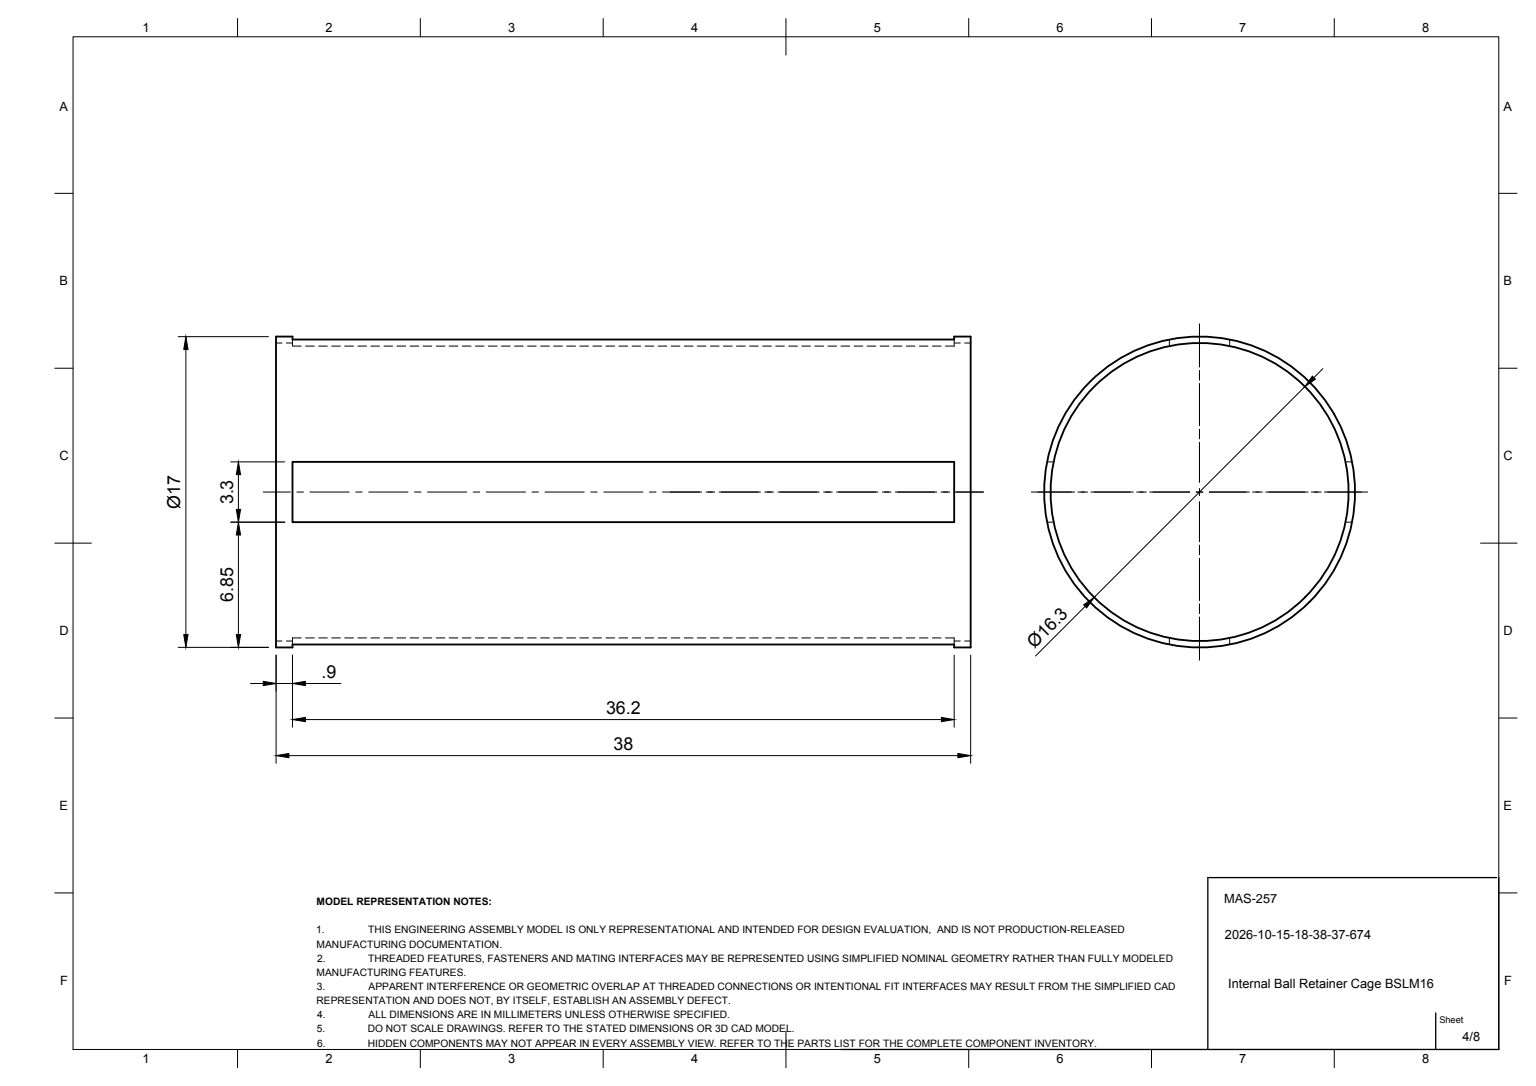
ISO-10303-21;
HEADER;
FILE_DESCRIPTION((''),'2;1');
FILE_NAME('Internal Ball Retainer Cage BSLM16.step','2026-10-05T22:33:56+05:00',(''),(''),'','','');
FILE_SCHEMA (('AUTOMOTIVE_DESIGN { 1 0 10303 214 3 1 1 }'));
ENDSEC;
DATA;
#10=MECHANICAL_DESIGN_GEOMETRIC_PRESENTATION_REPRESENTATION('',(#431),#16942);
#417=SHAPE_REPRESENTATION_RELATIONSHIP('SRR','None',#17021,#424) ;
#424=ADVANCED_BREP_SHAPE_REPRESENTATION('',(#438),#16937) ;
#431=STYLED_ITEM('',(#17065),#438) ;
#438=MANIFOLD_SOLID_BREP('Internal Ball Retainer Cage BSLM16',#8180) ;
#719=FACE_BOUND('',#1778,.T.) ;
#720=FACE_BOUND('',#1779,.T.) ;
#721=FACE_BOUND('',#1780,.T.) ;
#722=FACE_BOUND('',#1781,.T.) ;
#723=FACE_BOUND('',#1783,.T.) ;
#724=FACE_BOUND('',#1785,.T.) ;
#725=FACE_BOUND('',#1786,.T.) ;
#726=FACE_BOUND('',#1787,.T.) ;
#727=FACE_BOUND('',#1788,.T.) ;
#728=FACE_BOUND('',#1790,.T.) ;
#818=PLANE('',#8553) ;
#819=PLANE('',#8554) ;
#820=PLANE('',#8557) ;
#821=PLANE('',#8558) ;
#822=PLANE('',#8561) ;
#823=PLANE('',#8562) ;
#824=PLANE('',#8565) ;
#825=PLANE('',#8566) ;
#826=PLANE('',#8569) ;
#827=PLANE('',#8570) ;
#828=PLANE('',#8573) ;
#829=PLANE('',#8574) ;
#830=PLANE('',#8577) ;
#831=PLANE('',#8578) ;
#832=PLANE('',#8581) ;
#833=PLANE('',#8582) ;
#834=PLANE('',#8588) ;
#835=PLANE('',#8592) ;
#1016=CYLINDRICAL_SURFACE('',#8585,8.15) ;
#1017=CYLINDRICAL_SURFACE('',#8590,8.5) ;
#1286=FACE_OUTER_BOUND('',#1761,.T.) ;
#1287=FACE_OUTER_BOUND('',#1762,.T.) ;
#1288=FACE_OUTER_BOUND('',#1763,.T.) ;
#1289=FACE_OUTER_BOUND('',#1764,.T.) ;
#1290=FACE_OUTER_BOUND('',#1765,.T.) ;
#1291=FACE_OUTER_BOUND('',#1766,.T.) ;
#1292=FACE_OUTER_BOUND('',#1767,.T.) ;
#1293=FACE_OUTER_BOUND('',#1768,.T.) ;
#1294=FACE_OUTER_BOUND('',#1769,.T.) ;
#1295=FACE_OUTER_BOUND('',#1770,.T.) ;
#1296=FACE_OUTER_BOUND('',#1771,.T.) ;
#1297=FACE_OUTER_BOUND('',#1772,.T.) ;
#1298=FACE_OUTER_BOUND('',#1773,.T.) ;
#1299=FACE_OUTER_BOUND('',#1774,.T.) ;
#1300=FACE_OUTER_BOUND('',#1775,.T.) ;
#1301=FACE_OUTER_BOUND('',#1776,.T.) ;
#1302=FACE_OUTER_BOUND('',#1777,.T.) ;
#1303=FACE_OUTER_BOUND('',#1782,.T.) ;
#1304=FACE_OUTER_BOUND('',#1784,.T.) ;
#1305=FACE_OUTER_BOUND('',#1789,.T.) ;
#1761=EDGE_LOOP('',(#6517,#6518,#6519,#6520)) ;
#1762=EDGE_LOOP('',(#6521,#6522,#6523,#6524)) ;
#1763=EDGE_LOOP('',(#6525,#6526,#6527,#6528)) ;
#1764=EDGE_LOOP('',(#6529,#6530,#6531,#6532)) ;
#1765=EDGE_LOOP('',(#6533,#6534,#6535,#6536)) ;
#1766=EDGE_LOOP('',(#6537,#6538,#6539,#6540)) ;
#1767=EDGE_LOOP('',(#6541,#6542,#6543,#6544)) ;
#1768=EDGE_LOOP('',(#6545,#6546,#6547,#6548)) ;
#1769=EDGE_LOOP('',(#6549,#6550,#6551,#6552)) ;
#1770=EDGE_LOOP('',(#6553,#6554,#6555,#6556)) ;
#1771=EDGE_LOOP('',(#6557,#6558,#6559,#6560)) ;
#1772=EDGE_LOOP('',(#6561,#6562,#6563,#6564)) ;
#1773=EDGE_LOOP('',(#6565,#6566,#6567,#6568)) ;
#1774=EDGE_LOOP('',(#6569,#6570,#6571,#6572)) ;
#1775=EDGE_LOOP('',(#6573,#6574,#6575,#6576)) ;
#1776=EDGE_LOOP('',(#6577,#6578,#6579,#6580)) ;
#1777=EDGE_LOOP('',(#6581,#6582,#6583,#6584)) ;
#1778=EDGE_LOOP('',(#6585,#6586,#6587,#6588)) ;
#1779=EDGE_LOOP('',(#6589,#6590,#6591,#6592)) ;
#1780=EDGE_LOOP('',(#6593,#6594,#6595,#6596)) ;
#1781=EDGE_LOOP('',(#6597,#6598,#6599,#6600)) ;
#1782=EDGE_LOOP('',(#6601)) ;
#1783=EDGE_LOOP('',(#6602)) ;
#1784=EDGE_LOOP('',(#6603,#6604,#6605,#6606)) ;
#1785=EDGE_LOOP('',(#6607,#6608,#6609,#6610)) ;
#1786=EDGE_LOOP('',(#6611,#6612,#6613,#6614)) ;
#1787=EDGE_LOOP('',(#6615,#6616,#6617,#6618)) ;
#1788=EDGE_LOOP('',(#6619,#6620,#6621,#6622)) ;
#1789=EDGE_LOOP('',(#6623)) ;
#1790=EDGE_LOOP('',(#6624)) ;
#2253=LINE('',#13606,#2815) ;
#2254=LINE('',#13608,#2816) ;
#2255=LINE('',#13610,#2817) ;
#2256=LINE('',#13611,#2818) ;
#2257=LINE('',#13617,#2819) ;
#2258=LINE('',#13620,#2820) ;
#2259=LINE('',#13622,#2821) ;
#2260=LINE('',#13623,#2822) ;
#2261=LINE('',#13630,#2823) ;
#2262=LINE('',#13632,#2824) ;
#2263=LINE('',#13634,#2825) ;
#2264=LINE('',#13635,#2826) ;
#2265=LINE('',#13641,#2827) ;
#2266=LINE('',#13644,#2828) ;
#2267=LINE('',#13646,#2829) ;
#2268=LINE('',#13647,#2830) ;
#2269=LINE('',#13654,#2831) ;
#2270=LINE('',#13656,#2832) ;
#2271=LINE('',#13658,#2833) ;
#2272=LINE('',#13659,#2834) ;
#2273=LINE('',#13665,#2835) ;
#2274=LINE('',#13668,#2836) ;
#2275=LINE('',#13670,#2837) ;
#2276=LINE('',#13671,#2838) ;
#2277=LINE('',#13678,#2839) ;
#2278=LINE('',#13680,#2840) ;
#2279=LINE('',#13682,#2841) ;
#2280=LINE('',#13683,#2842) ;
#2281=LINE('',#13689,#2843) ;
#2282=LINE('',#13692,#2844) ;
#2283=LINE('',#13694,#2845) ;
#2284=LINE('',#13695,#2846) ;
#2285=LINE('',#13703,#2847) ;
#2286=LINE('',#13711,#2848) ;
#2815=VECTOR('',#9811,10.) ;
#2816=VECTOR('',#9812,10.) ;
#2817=VECTOR('',#9813,10.) ;
#2818=VECTOR('',#9814,10.) ;
#2819=VECTOR('',#9821,10.) ;
#2820=VECTOR('',#9824,10.) ;
#2821=VECTOR('',#9825,10.) ;
#2822=VECTOR('',#9826,10.) ;
#2823=VECTOR('',#9835,10.) ;
#2824=VECTOR('',#9836,10.) ;
#2825=VECTOR('',#9837,10.) ;
#2826=VECTOR('',#9838,10.) ;
#2827=VECTOR('',#9845,10.) ;
#2828=VECTOR('',#9848,10.) ;
#2829=VECTOR('',#9849,10.) ;
#2830=VECTOR('',#9850,10.) ;
#2831=VECTOR('',#9859,10.) ;
#2832=VECTOR('',#9860,10.) ;
#2833=VECTOR('',#9861,10.) ;
#2834=VECTOR('',#9862,10.) ;
#2835=VECTOR('',#9869,10.) ;
#2836=VECTOR('',#9872,10.) ;
#2837=VECTOR('',#9873,10.) ;
#2838=VECTOR('',#9874,10.) ;
#2839=VECTOR('',#9883,10.) ;
#2840=VECTOR('',#9884,10.) ;
#2841=VECTOR('',#9885,10.) ;
#2842=VECTOR('',#9886,10.) ;
#2843=VECTOR('',#9893,10.) ;
#2844=VECTOR('',#9896,10.) ;
#2845=VECTOR('',#9897,10.) ;
#2846=VECTOR('',#9898,10.) ;
#2847=VECTOR('',#9909,8.15) ;
#2848=VECTOR('',#9920,8.5) ;
#3253=CIRCLE('',#8555,8.15) ;
#3254=CIRCLE('',#8556,8.5) ;
#3255=CIRCLE('',#8559,8.15) ;
#3256=CIRCLE('',#8560,8.5) ;
#3257=CIRCLE('',#8563,8.15) ;
#3258=CIRCLE('',#8564,8.5) ;
#3259=CIRCLE('',#8567,8.15) ;
#3260=CIRCLE('',#8568,8.5) ;
#3261=CIRCLE('',#8571,8.15) ;
#3262=CIRCLE('',#8572,8.5) ;
#3263=CIRCLE('',#8575,8.15) ;
#3264=CIRCLE('',#8576,8.5) ;
#3265=CIRCLE('',#8579,8.15) ;
#3266=CIRCLE('',#8580,8.5) ;
#3267=CIRCLE('',#8583,8.15) ;
#3268=CIRCLE('',#8584,8.5) ;
#3269=CIRCLE('',#8586,8.15) ;
#3270=CIRCLE('',#8587,8.15) ;
#3271=CIRCLE('',#8589,8.5) ;
#3272=CIRCLE('',#8591,8.5) ;
#3783=VERTEX_POINT('',#13604) ;
#3784=VERTEX_POINT('',#13605) ;
#3785=VERTEX_POINT('',#13607) ;
#3786=VERTEX_POINT('',#13609) ;
#3787=VERTEX_POINT('',#13613) ;
#3788=VERTEX_POINT('',#13615) ;
#3789=VERTEX_POINT('',#13619) ;
#3790=VERTEX_POINT('',#13621) ;
#3791=VERTEX_POINT('',#13628) ;
#3792=VERTEX_POINT('',#13629) ;
#3793=VERTEX_POINT('',#13631) ;
#3794=VERTEX_POINT('',#13633) ;
#3795=VERTEX_POINT('',#13637) ;
#3796=VERTEX_POINT('',#13639) ;
#3797=VERTEX_POINT('',#13643) ;
#3798=VERTEX_POINT('',#13645) ;
#3799=VERTEX_POINT('',#13652) ;
#3800=VERTEX_POINT('',#13653) ;
#3801=VERTEX_POINT('',#13655) ;
#3802=VERTEX_POINT('',#13657) ;
#3803=VERTEX_POINT('',#13661) ;
#3804=VERTEX_POINT('',#13663) ;
#3805=VERTEX_POINT('',#13667) ;
#3806=VERTEX_POINT('',#13669) ;
#3807=VERTEX_POINT('',#13676) ;
#3808=VERTEX_POINT('',#13677) ;
#3809=VERTEX_POINT('',#13679) ;
#3810=VERTEX_POINT('',#13681) ;
#3811=VERTEX_POINT('',#13685) ;
#3812=VERTEX_POINT('',#13687) ;
#3813=VERTEX_POINT('',#13691) ;
#3814=VERTEX_POINT('',#13693) ;
#3815=VERTEX_POINT('',#13700) ;
#3816=VERTEX_POINT('',#13702) ;
#3817=VERTEX_POINT('',#13706) ;
#3818=VERTEX_POINT('',#13709) ;
#4756=EDGE_CURVE('',#3783,#3784,#2253,.T.) ;
#4757=EDGE_CURVE('',#3783,#3785,#2254,.T.) ;
#4758=EDGE_CURVE('',#3786,#3785,#2255,.T.) ;
#4759=EDGE_CURVE('',#3786,#3784,#2256,.T.) ;
#4760=EDGE_CURVE('',#3784,#3787,#3253,.T.) ;
#4761=EDGE_CURVE('',#3788,#3786,#3254,.T.) ;
#4762=EDGE_CURVE('',#3787,#3788,#2257,.T.) ;
#4763=EDGE_CURVE('',#3787,#3789,#2258,.T.) ;
#4764=EDGE_CURVE('',#3790,#3788,#2259,.T.) ;
#4765=EDGE_CURVE('',#3790,#3789,#2260,.T.) ;
#4766=EDGE_CURVE('',#3789,#3783,#3255,.T.) ;
#4767=EDGE_CURVE('',#3785,#3790,#3256,.T.) ;
#4768=EDGE_CURVE('',#3791,#3792,#2261,.T.) ;
#4769=EDGE_CURVE('',#3791,#3793,#2262,.T.) ;
#4770=EDGE_CURVE('',#3794,#3793,#2263,.T.) ;
#4771=EDGE_CURVE('',#3794,#3792,#2264,.T.) ;
#4772=EDGE_CURVE('',#3792,#3795,#3257,.T.) ;
#4773=EDGE_CURVE('',#3796,#3794,#3258,.T.) ;
#4774=EDGE_CURVE('',#3795,#3796,#2265,.T.) ;
#4775=EDGE_CURVE('',#3795,#3797,#2266,.T.) ;
#4776=EDGE_CURVE('',#3798,#3796,#2267,.T.) ;
#4777=EDGE_CURVE('',#3798,#3797,#2268,.T.) ;
#4778=EDGE_CURVE('',#3797,#3791,#3259,.T.) ;
#4779=EDGE_CURVE('',#3793,#3798,#3260,.T.) ;
#4780=EDGE_CURVE('',#3799,#3800,#2269,.T.) ;
#4781=EDGE_CURVE('',#3799,#3801,#2270,.T.) ;
#4782=EDGE_CURVE('',#3802,#3801,#2271,.T.) ;
#4783=EDGE_CURVE('',#3802,#3800,#2272,.T.) ;
#4784=EDGE_CURVE('',#3800,#3803,#3261,.T.) ;
#4785=EDGE_CURVE('',#3804,#3802,#3262,.T.) ;
#4786=EDGE_CURVE('',#3803,#3804,#2273,.T.) ;
#4787=EDGE_CURVE('',#3803,#3805,#2274,.T.) ;
#4788=EDGE_CURVE('',#3806,#3804,#2275,.T.) ;
#4789=EDGE_CURVE('',#3806,#3805,#2276,.T.) ;
#4790=EDGE_CURVE('',#3805,#3799,#3263,.T.) ;
#4791=EDGE_CURVE('',#3801,#3806,#3264,.T.) ;
#4792=EDGE_CURVE('',#3807,#3808,#2277,.T.) ;
#4793=EDGE_CURVE('',#3807,#3809,#2278,.T.) ;
#4794=EDGE_CURVE('',#3810,#3809,#2279,.T.) ;
#4795=EDGE_CURVE('',#3810,#3808,#2280,.T.) ;
#4796=EDGE_CURVE('',#3808,#3811,#3265,.T.) ;
#4797=EDGE_CURVE('',#3812,#3810,#3266,.T.) ;
#4798=EDGE_CURVE('',#3811,#3812,#2281,.T.) ;
#4799=EDGE_CURVE('',#3811,#3813,#2282,.T.) ;
#4800=EDGE_CURVE('',#3814,#3812,#2283,.T.) ;
#4801=EDGE_CURVE('',#3814,#3813,#2284,.T.) ;
#4802=EDGE_CURVE('',#3813,#3807,#3267,.T.) ;
#4803=EDGE_CURVE('',#3809,#3814,#3268,.T.) ;
#4804=EDGE_CURVE('',#3815,#3815,#3269,.T.) ;
#4805=EDGE_CURVE('',#3815,#3816,#2285,.T.) ;
#4806=EDGE_CURVE('',#3816,#3816,#3270,.T.) ;
#4807=EDGE_CURVE('',#3817,#3817,#3271,.T.) ;
#4808=EDGE_CURVE('',#3818,#3818,#3272,.T.) ;
#4809=EDGE_CURVE('',#3818,#3817,#2286,.T.) ;
#6517=ORIENTED_EDGE('',*,*,#4756,.F.) ;
#6518=ORIENTED_EDGE('',*,*,#4757,.T.) ;
#6519=ORIENTED_EDGE('',*,*,#4758,.F.) ;
#6520=ORIENTED_EDGE('',*,*,#4759,.T.) ;
#6521=ORIENTED_EDGE('',*,*,#4760,.F.) ;
#6522=ORIENTED_EDGE('',*,*,#4759,.F.) ;
#6523=ORIENTED_EDGE('',*,*,#4761,.F.) ;
#6524=ORIENTED_EDGE('',*,*,#4762,.F.) ;
#6525=ORIENTED_EDGE('',*,*,#4763,.F.) ;
#6526=ORIENTED_EDGE('',*,*,#4762,.T.) ;
#6527=ORIENTED_EDGE('',*,*,#4764,.F.) ;
#6528=ORIENTED_EDGE('',*,*,#4765,.T.) ;
#6529=ORIENTED_EDGE('',*,*,#4766,.F.) ;
#6530=ORIENTED_EDGE('',*,*,#4765,.F.) ;
#6531=ORIENTED_EDGE('',*,*,#4767,.F.) ;
#6532=ORIENTED_EDGE('',*,*,#4757,.F.) ;
#6533=ORIENTED_EDGE('',*,*,#4768,.F.) ;
#6534=ORIENTED_EDGE('',*,*,#4769,.T.) ;
#6535=ORIENTED_EDGE('',*,*,#4770,.F.) ;
#6536=ORIENTED_EDGE('',*,*,#4771,.T.) ;
#6537=ORIENTED_EDGE('',*,*,#4772,.F.) ;
#6538=ORIENTED_EDGE('',*,*,#4771,.F.) ;
#6539=ORIENTED_EDGE('',*,*,#4773,.F.) ;
#6540=ORIENTED_EDGE('',*,*,#4774,.F.) ;
#6541=ORIENTED_EDGE('',*,*,#4775,.F.) ;
#6542=ORIENTED_EDGE('',*,*,#4774,.T.) ;
#6543=ORIENTED_EDGE('',*,*,#4776,.F.) ;
#6544=ORIENTED_EDGE('',*,*,#4777,.T.) ;
#6545=ORIENTED_EDGE('',*,*,#4778,.F.) ;
#6546=ORIENTED_EDGE('',*,*,#4777,.F.) ;
#6547=ORIENTED_EDGE('',*,*,#4779,.F.) ;
#6548=ORIENTED_EDGE('',*,*,#4769,.F.) ;
#6549=ORIENTED_EDGE('',*,*,#4780,.F.) ;
#6550=ORIENTED_EDGE('',*,*,#4781,.T.) ;
#6551=ORIENTED_EDGE('',*,*,#4782,.F.) ;
#6552=ORIENTED_EDGE('',*,*,#4783,.T.) ;
#6553=ORIENTED_EDGE('',*,*,#4784,.F.) ;
#6554=ORIENTED_EDGE('',*,*,#4783,.F.) ;
#6555=ORIENTED_EDGE('',*,*,#4785,.F.) ;
#6556=ORIENTED_EDGE('',*,*,#4786,.F.) ;
#6557=ORIENTED_EDGE('',*,*,#4787,.F.) ;
#6558=ORIENTED_EDGE('',*,*,#4786,.T.) ;
#6559=ORIENTED_EDGE('',*,*,#4788,.F.) ;
#6560=ORIENTED_EDGE('',*,*,#4789,.T.) ;
#6561=ORIENTED_EDGE('',*,*,#4790,.F.) ;
#6562=ORIENTED_EDGE('',*,*,#4789,.F.) ;
#6563=ORIENTED_EDGE('',*,*,#4791,.F.) ;
#6564=ORIENTED_EDGE('',*,*,#4781,.F.) ;
#6565=ORIENTED_EDGE('',*,*,#4792,.F.) ;
#6566=ORIENTED_EDGE('',*,*,#4793,.T.) ;
#6567=ORIENTED_EDGE('',*,*,#4794,.F.) ;
#6568=ORIENTED_EDGE('',*,*,#4795,.T.) ;
#6569=ORIENTED_EDGE('',*,*,#4796,.F.) ;
#6570=ORIENTED_EDGE('',*,*,#4795,.F.) ;
#6571=ORIENTED_EDGE('',*,*,#4797,.F.) ;
#6572=ORIENTED_EDGE('',*,*,#4798,.F.) ;
#6573=ORIENTED_EDGE('',*,*,#4799,.F.) ;
#6574=ORIENTED_EDGE('',*,*,#4798,.T.) ;
#6575=ORIENTED_EDGE('',*,*,#4800,.F.) ;
#6576=ORIENTED_EDGE('',*,*,#4801,.T.) ;
#6577=ORIENTED_EDGE('',*,*,#4802,.F.) ;
#6578=ORIENTED_EDGE('',*,*,#4801,.F.) ;
#6579=ORIENTED_EDGE('',*,*,#4803,.F.) ;
#6580=ORIENTED_EDGE('',*,*,#4793,.F.) ;
#6581=ORIENTED_EDGE('',*,*,#4804,.T.) ;
#6582=ORIENTED_EDGE('',*,*,#4805,.T.) ;
#6583=ORIENTED_EDGE('',*,*,#4806,.F.) ;
#6584=ORIENTED_EDGE('',*,*,#4805,.F.) ;
#6585=ORIENTED_EDGE('',*,*,#4763,.T.) ;
#6586=ORIENTED_EDGE('',*,*,#4766,.T.) ;
#6587=ORIENTED_EDGE('',*,*,#4756,.T.) ;
#6588=ORIENTED_EDGE('',*,*,#4760,.T.) ;
#6589=ORIENTED_EDGE('',*,*,#4775,.T.) ;
#6590=ORIENTED_EDGE('',*,*,#4778,.T.) ;
#6591=ORIENTED_EDGE('',*,*,#4768,.T.) ;
#6592=ORIENTED_EDGE('',*,*,#4772,.T.) ;
#6593=ORIENTED_EDGE('',*,*,#4787,.T.) ;
#6594=ORIENTED_EDGE('',*,*,#4790,.T.) ;
#6595=ORIENTED_EDGE('',*,*,#4780,.T.) ;
#6596=ORIENTED_EDGE('',*,*,#4784,.T.) ;
#6597=ORIENTED_EDGE('',*,*,#4799,.T.) ;
#6598=ORIENTED_EDGE('',*,*,#4802,.T.) ;
#6599=ORIENTED_EDGE('',*,*,#4792,.T.) ;
#6600=ORIENTED_EDGE('',*,*,#4796,.T.) ;
#6601=ORIENTED_EDGE('',*,*,#4807,.F.) ;
#6602=ORIENTED_EDGE('',*,*,#4806,.T.) ;
#6603=ORIENTED_EDGE('',*,*,#4808,.F.) ;
#6604=ORIENTED_EDGE('',*,*,#4809,.T.) ;
#6605=ORIENTED_EDGE('',*,*,#4807,.T.) ;
#6606=ORIENTED_EDGE('',*,*,#4809,.F.) ;
#6607=ORIENTED_EDGE('',*,*,#4764,.T.) ;
#6608=ORIENTED_EDGE('',*,*,#4761,.T.) ;
#6609=ORIENTED_EDGE('',*,*,#4758,.T.) ;
#6610=ORIENTED_EDGE('',*,*,#4767,.T.) ;
#6611=ORIENTED_EDGE('',*,*,#4776,.T.) ;
#6612=ORIENTED_EDGE('',*,*,#4773,.T.) ;
#6613=ORIENTED_EDGE('',*,*,#4770,.T.) ;
#6614=ORIENTED_EDGE('',*,*,#4779,.T.) ;
#6615=ORIENTED_EDGE('',*,*,#4788,.T.) ;
#6616=ORIENTED_EDGE('',*,*,#4785,.T.) ;
#6617=ORIENTED_EDGE('',*,*,#4782,.T.) ;
#6618=ORIENTED_EDGE('',*,*,#4791,.T.) ;
#6619=ORIENTED_EDGE('',*,*,#4800,.T.) ;
#6620=ORIENTED_EDGE('',*,*,#4797,.T.) ;
#6621=ORIENTED_EDGE('',*,*,#4794,.T.) ;
#6622=ORIENTED_EDGE('',*,*,#4803,.T.) ;
#6623=ORIENTED_EDGE('',*,*,#4808,.T.) ;
#6624=ORIENTED_EDGE('',*,*,#4804,.F.) ;
#7961=ADVANCED_FACE('',(#1286),#818,.F.) ;
#7962=ADVANCED_FACE('',(#1287),#819,.F.) ;
#7963=ADVANCED_FACE('',(#1288),#820,.F.) ;
#7964=ADVANCED_FACE('',(#1289),#821,.T.) ;
#7965=ADVANCED_FACE('',(#1290),#822,.F.) ;
#7966=ADVANCED_FACE('',(#1291),#823,.F.) ;
#7967=ADVANCED_FACE('',(#1292),#824,.F.) ;
#7968=ADVANCED_FACE('',(#1293),#825,.T.) ;
#7969=ADVANCED_FACE('',(#1294),#826,.F.) ;
#7970=ADVANCED_FACE('',(#1295),#827,.F.) ;
#7971=ADVANCED_FACE('',(#1296),#828,.F.) ;
#7972=ADVANCED_FACE('',(#1297),#829,.T.) ;
#7973=ADVANCED_FACE('',(#1298),#830,.F.) ;
#7974=ADVANCED_FACE('',(#1299),#831,.F.) ;
#7975=ADVANCED_FACE('',(#1300),#832,.F.) ;
#7976=ADVANCED_FACE('',(#1301),#833,.T.) ;
#7977=ADVANCED_FACE('',(#1302,#719,#720,#721,#722),#1016,.F.) ;
#7978=ADVANCED_FACE('',(#1303,#723),#834,.T.) ;
#7979=ADVANCED_FACE('',(#1304,#724,#725,#726,#727),#1017,.T.) ;
#7980=ADVANCED_FACE('',(#1305,#728),#835,.T.) ;
#8180=CLOSED_SHELL('',(#7961,#7962,#7963,#7964,#7965,#7966,#7967,#7968,
#7969,#7970,#7971,#7972,#7973,#7974,#7975,#7976,#7977,#7978,#7979,#7980)) ;
#8552=AXIS2_PLACEMENT_3D('',#13602,#9807,#9808) ;
#8553=AXIS2_PLACEMENT_3D('',#13603,#9809,#9810) ;
#8554=AXIS2_PLACEMENT_3D('',#13612,#9815,#9816) ;
#8555=AXIS2_PLACEMENT_3D('',#13614,#9817,#9818) ;
#8556=AXIS2_PLACEMENT_3D('',#13616,#9819,#9820) ;
#8557=AXIS2_PLACEMENT_3D('',#13618,#9822,#9823) ;
#8558=AXIS2_PLACEMENT_3D('',#13624,#9827,#9828) ;
#8559=AXIS2_PLACEMENT_3D('',#13625,#9829,#9830) ;
#8560=AXIS2_PLACEMENT_3D('',#13626,#9831,#9832) ;
#8561=AXIS2_PLACEMENT_3D('',#13627,#9833,#9834) ;
#8562=AXIS2_PLACEMENT_3D('',#13636,#9839,#9840) ;
#8563=AXIS2_PLACEMENT_3D('',#13638,#9841,#9842) ;
#8564=AXIS2_PLACEMENT_3D('',#13640,#9843,#9844) ;
#8565=AXIS2_PLACEMENT_3D('',#13642,#9846,#9847) ;
#8566=AXIS2_PLACEMENT_3D('',#13648,#9851,#9852) ;
#8567=AXIS2_PLACEMENT_3D('',#13649,#9853,#9854) ;
#8568=AXIS2_PLACEMENT_3D('',#13650,#9855,#9856) ;
#8569=AXIS2_PLACEMENT_3D('',#13651,#9857,#9858) ;
#8570=AXIS2_PLACEMENT_3D('',#13660,#9863,#9864) ;
#8571=AXIS2_PLACEMENT_3D('',#13662,#9865,#9866) ;
#8572=AXIS2_PLACEMENT_3D('',#13664,#9867,#9868) ;
#8573=AXIS2_PLACEMENT_3D('',#13666,#9870,#9871) ;
#8574=AXIS2_PLACEMENT_3D('',#13672,#9875,#9876) ;
#8575=AXIS2_PLACEMENT_3D('',#13673,#9877,#9878) ;
#8576=AXIS2_PLACEMENT_3D('',#13674,#9879,#9880) ;
#8577=AXIS2_PLACEMENT_3D('',#13675,#9881,#9882) ;
#8578=AXIS2_PLACEMENT_3D('',#13684,#9887,#9888) ;
#8579=AXIS2_PLACEMENT_3D('',#13686,#9889,#9890) ;
#8580=AXIS2_PLACEMENT_3D('',#13688,#9891,#9892) ;
#8581=AXIS2_PLACEMENT_3D('',#13690,#9894,#9895) ;
#8582=AXIS2_PLACEMENT_3D('',#13696,#9899,#9900) ;
#8583=AXIS2_PLACEMENT_3D('',#13697,#9901,#9902) ;
#8584=AXIS2_PLACEMENT_3D('',#13698,#9903,#9904) ;
#8585=AXIS2_PLACEMENT_3D('',#13699,#9905,#9906) ;
#8586=AXIS2_PLACEMENT_3D('',#13701,#9907,#9908) ;
#8587=AXIS2_PLACEMENT_3D('',#13704,#9910,#9911) ;
#8588=AXIS2_PLACEMENT_3D('',#13705,#9912,#9913) ;
#8589=AXIS2_PLACEMENT_3D('',#13707,#9914,#9915) ;
#8590=AXIS2_PLACEMENT_3D('',#13708,#9916,#9917) ;
#8591=AXIS2_PLACEMENT_3D('',#13710,#9918,#9919) ;
#8592=AXIS2_PLACEMENT_3D('',#13712,#9921,#9922) ;
#9807=DIRECTION('axis',(0.,0.,1.)) ;
#9808=DIRECTION('refdir',(1.,0.,0.)) ;
#9809=DIRECTION('center_axis',(0.,0.707106781186547,-0.707106781186548)) ;
#9810=DIRECTION('ref_axis',(0.,0.707106781186548,0.707106781186547)) ;
#9811=DIRECTION('',(1.,0.,0.)) ;
#9812=DIRECTION('',(0.,-0.707106781186548,-0.707106781186547)) ;
#9813=DIRECTION('',(-1.,0.,0.)) ;
#9814=DIRECTION('',(0.,0.707106781186548,0.707106781186547)) ;
#9815=DIRECTION('center_axis',(1.,0.,0.)) ;
#9816=DIRECTION('ref_axis',(0.,0.,-1.)) ;
#9817=DIRECTION('center_axis',(-1.,0.,0.)) ;
#9818=DIRECTION('ref_axis',(0.,1.,0.)) ;
#9819=DIRECTION('center_axis',(1.,0.,0.)) ;
#9820=DIRECTION('ref_axis',(0.,1.,0.)) ;
#9821=DIRECTION('',(0.,-0.707106781186547,-0.707106781186548)) ;
#9822=DIRECTION('center_axis',(0.,-0.707106781186548,0.707106781186547)) ;
#9823=DIRECTION('ref_axis',(0.,-0.707106781186547,-0.707106781186548)) ;
#9824=DIRECTION('',(-1.,0.,0.)) ;
#9825=DIRECTION('',(1.,0.,0.)) ;
#9826=DIRECTION('',(0.,0.707106781186547,0.707106781186548)) ;
#9827=DIRECTION('center_axis',(1.,0.,0.)) ;
#9828=DIRECTION('ref_axis',(0.,0.,-1.)) ;
#9829=DIRECTION('center_axis',(1.,0.,0.)) ;
#9830=DIRECTION('ref_axis',(0.,1.,0.)) ;
#9831=DIRECTION('center_axis',(-1.,0.,0.)) ;
#9832=DIRECTION('ref_axis',(0.,1.,0.)) ;
#9833=DIRECTION('center_axis',(0.,0.707106781186549,0.707106781186546)) ;
#9834=DIRECTION('ref_axis',(0.,-0.707106781186546,0.707106781186549)) ;
#9835=DIRECTION('',(1.,0.,0.)) ;
#9836=DIRECTION('',(0.,0.707106781186546,-0.707106781186549)) ;
#9837=DIRECTION('',(-1.,0.,0.)) ;
#9838=DIRECTION('',(0.,-0.707106781186546,0.707106781186549)) ;
#9839=DIRECTION('center_axis',(1.,0.,0.)) ;
#9840=DIRECTION('ref_axis',(0.,0.,-1.)) ;
#9841=DIRECTION('center_axis',(-1.,0.,0.)) ;
#9842=DIRECTION('ref_axis',(0.,1.,0.)) ;
#9843=DIRECTION('center_axis',(1.,0.,0.)) ;
#9844=DIRECTION('ref_axis',(0.,1.,0.)) ;
#9845=DIRECTION('',(0.,0.707106781186548,-0.707106781186547)) ;
#9846=DIRECTION('center_axis',(0.,-0.707106781186547,-0.707106781186548)) ;
#9847=DIRECTION('ref_axis',(0.,0.707106781186548,-0.707106781186547)) ;
#9848=DIRECTION('',(-1.,0.,0.)) ;
#9849=DIRECTION('',(1.,0.,0.)) ;
#9850=DIRECTION('',(0.,-0.707106781186548,0.707106781186547)) ;
#9851=DIRECTION('center_axis',(1.,0.,0.)) ;
#9852=DIRECTION('ref_axis',(0.,0.,-1.)) ;
#9853=DIRECTION('center_axis',(1.,0.,0.)) ;
#9854=DIRECTION('ref_axis',(0.,1.,0.)) ;
#9855=DIRECTION('center_axis',(-1.,0.,0.)) ;
#9856=DIRECTION('ref_axis',(0.,1.,0.)) ;
#9857=DIRECTION('center_axis',(0.,-0.707106781186546,0.707106781186549)) ;
#9858=DIRECTION('ref_axis',(0.,-0.707106781186549,-0.707106781186546)) ;
#9859=DIRECTION('',(1.,0.,0.)) ;
#9860=DIRECTION('',(0.,0.707106781186549,0.707106781186546)) ;
#9861=DIRECTION('',(-1.,0.,0.)) ;
#9862=DIRECTION('',(0.,-0.707106781186549,-0.707106781186546)) ;
#9863=DIRECTION('center_axis',(1.,0.,0.)) ;
#9864=DIRECTION('ref_axis',(0.,0.,-1.)) ;
#9865=DIRECTION('center_axis',(-1.,0.,0.)) ;
#9866=DIRECTION('ref_axis',(0.,1.,0.)) ;
#9867=DIRECTION('center_axis',(1.,0.,0.)) ;
#9868=DIRECTION('ref_axis',(0.,1.,0.)) ;
#9869=DIRECTION('',(0.,0.707106781186546,0.707106781186549)) ;
#9870=DIRECTION('center_axis',(0.,0.707106781186549,-0.707106781186546)) ;
#9871=DIRECTION('ref_axis',(0.,0.707106781186546,0.707106781186549)) ;
#9872=DIRECTION('',(-1.,0.,0.)) ;
#9873=DIRECTION('',(1.,0.,0.)) ;
#9874=DIRECTION('',(0.,-0.707106781186546,-0.707106781186549)) ;
#9875=DIRECTION('center_axis',(1.,0.,0.)) ;
#9876=DIRECTION('ref_axis',(0.,0.,-1.)) ;
#9877=DIRECTION('center_axis',(1.,0.,0.)) ;
#9878=DIRECTION('ref_axis',(0.,1.,0.)) ;
#9879=DIRECTION('center_axis',(-1.,0.,0.)) ;
#9880=DIRECTION('ref_axis',(0.,1.,0.)) ;
#9881=DIRECTION('center_axis',(0.,-0.707106781186548,-0.707106781186547)) ;
#9882=DIRECTION('ref_axis',(0.,0.707106781186547,-0.707106781186548)) ;
#9883=DIRECTION('',(1.,0.,0.)) ;
#9884=DIRECTION('',(0.,-0.707106781186547,0.707106781186548)) ;
#9885=DIRECTION('',(-1.,0.,0.)) ;
#9886=DIRECTION('',(0.,0.707106781186547,-0.707106781186548)) ;
#9887=DIRECTION('center_axis',(1.,0.,0.)) ;
#9888=DIRECTION('ref_axis',(0.,0.,-1.)) ;
#9889=DIRECTION('center_axis',(-1.,0.,0.)) ;
#9890=DIRECTION('ref_axis',(0.,1.,0.)) ;
#9891=DIRECTION('center_axis',(1.,0.,0.)) ;
#9892=DIRECTION('ref_axis',(0.,1.,0.)) ;
#9893=DIRECTION('',(0.,-0.707106781186546,0.707106781186549)) ;
#9894=DIRECTION('center_axis',(0.,0.707106781186549,0.707106781186546)) ;
#9895=DIRECTION('ref_axis',(0.,-0.707106781186546,0.707106781186549)) ;
#9896=DIRECTION('',(-1.,0.,0.)) ;
#9897=DIRECTION('',(1.,0.,0.)) ;
#9898=DIRECTION('',(0.,0.707106781186546,-0.707106781186549)) ;
#9899=DIRECTION('center_axis',(1.,0.,0.)) ;
#9900=DIRECTION('ref_axis',(0.,0.,-1.)) ;
#9901=DIRECTION('center_axis',(1.,0.,0.)) ;
#9902=DIRECTION('ref_axis',(0.,1.,0.)) ;
#9903=DIRECTION('center_axis',(-1.,0.,0.)) ;
#9904=DIRECTION('ref_axis',(0.,1.,0.)) ;
#9905=DIRECTION('center_axis',(1.,0.,0.)) ;
#9906=DIRECTION('ref_axis',(0.,1.,0.)) ;
#9907=DIRECTION('center_axis',(1.,0.,0.)) ;
#9908=DIRECTION('ref_axis',(0.,0.,-1.)) ;
#9909=DIRECTION('',(-1.,0.,0.)) ;
#9910=DIRECTION('center_axis',(1.,0.,0.)) ;
#9911=DIRECTION('ref_axis',(0.,0.,-1.)) ;
#9912=DIRECTION('center_axis',(-1.,0.,0.)) ;
#9913=DIRECTION('ref_axis',(0.,0.,1.)) ;
#9914=DIRECTION('center_axis',(1.,0.,0.)) ;
#9915=DIRECTION('ref_axis',(0.,0.,-1.)) ;
#9916=DIRECTION('center_axis',(1.,0.,0.)) ;
#9917=DIRECTION('ref_axis',(0.,1.,0.)) ;
#9918=DIRECTION('center_axis',(1.,0.,0.)) ;
#9919=DIRECTION('ref_axis',(0.,0.,-1.)) ;
#9920=DIRECTION('',(-1.,0.,0.)) ;
#9921=DIRECTION('center_axis',(1.,0.,0.)) ;
#9922=DIRECTION('ref_axis',(0.,0.,-1.)) ;
#13602=CARTESIAN_POINT('',(0.,0.,0.)) ;
#13603=CARTESIAN_POINT('Origin',(33.9,20.3027651582789,17.9693127803633)) ;
#13604=CARTESIAN_POINT('',(33.9,21.0231457651488,18.6896933872332)) ;
#13605=CARTESIAN_POINT('',(70.1,21.0231457651488,18.6896933872332)) ;
#13606=CARTESIAN_POINT('',(52.,21.0231457651488,18.6896933872332)) ;
#13607=CARTESIAN_POINT('',(33.9,20.7706469832483,18.4371946053327)) ;
#13608=CARTESIAN_POINT('',(33.9,21.29271465194,18.9592622740244)) ;
#13609=CARTESIAN_POINT('',(70.1,20.7706469832483,18.4371946053327)) ;
#13610=CARTESIAN_POINT('',(52.,20.7706469832483,18.4371946053327)) ;
#13611=CARTESIAN_POINT('',(70.1,21.29271465194,18.9592622740244)) ;
#13612=CARTESIAN_POINT('Origin',(70.1,19.6310137161517,19.6310137161517)) ;
#13613=CARTESIAN_POINT('',(70.1,18.6896933872332,21.0231457651488)) ;
#13614=CARTESIAN_POINT('Origin',(70.1,25.5,25.5)) ;
#13615=CARTESIAN_POINT('',(70.1,18.4371946053327,20.7706469832483)) ;
#13616=CARTESIAN_POINT('Origin',(70.1,25.5,25.5)) ;
#13617=CARTESIAN_POINT('',(70.1,17.9693127803633,20.3027651582789)) ;
#13618=CARTESIAN_POINT('Origin',(33.9,18.9592622740244,21.29271465194)) ;
#13619=CARTESIAN_POINT('',(33.9,18.6896933872332,21.0231457651488)) ;
#13620=CARTESIAN_POINT('',(52.,18.6896933872332,21.0231457651488)) ;
#13621=CARTESIAN_POINT('',(33.9,18.4371946053327,20.7706469832483)) ;
#13622=CARTESIAN_POINT('',(52.,18.4371946053327,20.7706469832483)) ;
#13623=CARTESIAN_POINT('',(33.9,17.9693127803633,20.3027651582789)) ;
#13624=CARTESIAN_POINT('Origin',(33.9,19.6310137161517,19.6310137161517)) ;
#13625=CARTESIAN_POINT('Origin',(33.9,25.5,25.5)) ;
#13626=CARTESIAN_POINT('Origin',(33.9,25.5,25.5)) ;
#13627=CARTESIAN_POINT('Origin',(33.9,33.0306872196367,20.3027651582789)) ;
#13628=CARTESIAN_POINT('',(33.9,32.3103066127668,21.0231457651488)) ;
#13629=CARTESIAN_POINT('',(70.1,32.3103066127668,21.0231457651488)) ;
#13630=CARTESIAN_POINT('',(52.,32.3103066127668,21.0231457651488)) ;
#13631=CARTESIAN_POINT('',(33.9,32.5628053946673,20.7706469832483)) ;
#13632=CARTESIAN_POINT('',(33.9,32.0407377259756,21.29271465194)) ;
#13633=CARTESIAN_POINT('',(70.1,32.5628053946673,20.7706469832483)) ;
#13634=CARTESIAN_POINT('',(52.,32.5628053946673,20.7706469832483)) ;
#13635=CARTESIAN_POINT('',(70.1,32.0407377259756,21.29271465194)) ;
#13636=CARTESIAN_POINT('Origin',(70.1,31.3689862838483,19.6310137161517)) ;
#13637=CARTESIAN_POINT('',(70.1,29.9768542348512,18.6896933872332)) ;
#13638=CARTESIAN_POINT('Origin',(70.1,25.5,25.5)) ;
#13639=CARTESIAN_POINT('',(70.1,30.2293530167517,18.4371946053327)) ;
#13640=CARTESIAN_POINT('Origin',(70.1,25.5,25.5)) ;
#13641=CARTESIAN_POINT('',(70.1,30.6972348417211,17.9693127803633)) ;
#13642=CARTESIAN_POINT('Origin',(33.9,29.70728534806,18.9592622740244)) ;
#13643=CARTESIAN_POINT('',(33.9,29.9768542348512,18.6896933872332)) ;
#13644=CARTESIAN_POINT('',(52.,29.9768542348512,18.6896933872332)) ;
#13645=CARTESIAN_POINT('',(33.9,30.2293530167517,18.4371946053327)) ;
#13646=CARTESIAN_POINT('',(52.,30.2293530167517,18.4371946053327)) ;
#13647=CARTESIAN_POINT('',(33.9,30.6972348417211,17.9693127803633)) ;
#13648=CARTESIAN_POINT('Origin',(33.9,31.3689862838483,19.6310137161517)) ;
#13649=CARTESIAN_POINT('Origin',(33.9,25.5,25.5)) ;
#13650=CARTESIAN_POINT('Origin',(33.9,25.5,25.5)) ;
#13651=CARTESIAN_POINT('Origin',(33.9,30.6972348417211,33.0306872196367)) ;
#13652=CARTESIAN_POINT('',(33.9,29.9768542348512,32.3103066127668)) ;
#13653=CARTESIAN_POINT('',(70.1,29.9768542348512,32.3103066127668)) ;
#13654=CARTESIAN_POINT('',(52.,29.9768542348512,32.3103066127668)) ;
#13655=CARTESIAN_POINT('',(33.9,30.2293530167517,32.5628053946673)) ;
#13656=CARTESIAN_POINT('',(33.9,29.70728534806,32.0407377259756)) ;
#13657=CARTESIAN_POINT('',(70.1,30.2293530167517,32.5628053946673)) ;
#13658=CARTESIAN_POINT('',(52.,30.2293530167517,32.5628053946673)) ;
#13659=CARTESIAN_POINT('',(70.1,29.70728534806,32.0407377259756)) ;
#13660=CARTESIAN_POINT('Origin',(70.1,31.3689862838483,31.3689862838483)) ;
#13661=CARTESIAN_POINT('',(70.1,32.3103066127668,29.9768542348512)) ;
#13662=CARTESIAN_POINT('Origin',(70.1,25.5,25.5)) ;
#13663=CARTESIAN_POINT('',(70.1,32.5628053946673,30.2293530167517)) ;
#13664=CARTESIAN_POINT('Origin',(70.1,25.5,25.5)) ;
#13665=CARTESIAN_POINT('',(70.1,33.0306872196367,30.6972348417211)) ;
#13666=CARTESIAN_POINT('Origin',(33.9,32.0407377259756,29.70728534806)) ;
#13667=CARTESIAN_POINT('',(33.9,32.3103066127668,29.9768542348512)) ;
#13668=CARTESIAN_POINT('',(52.,32.3103066127668,29.9768542348512)) ;
#13669=CARTESIAN_POINT('',(33.9,32.5628053946673,30.2293530167517)) ;
#13670=CARTESIAN_POINT('',(52.,32.5628053946673,30.2293530167517)) ;
#13671=CARTESIAN_POINT('',(33.9,33.0306872196367,30.6972348417211)) ;
#13672=CARTESIAN_POINT('Origin',(33.9,31.3689862838483,31.3689862838483)) ;
#13673=CARTESIAN_POINT('Origin',(33.9,25.5,25.5)) ;
#13674=CARTESIAN_POINT('Origin',(33.9,25.5,25.5)) ;
#13675=CARTESIAN_POINT('Origin',(33.9,17.9693127803633,30.6972348417211)) ;
#13676=CARTESIAN_POINT('',(33.9,18.6896933872332,29.9768542348512)) ;
#13677=CARTESIAN_POINT('',(70.1,18.6896933872332,29.9768542348512)) ;
#13678=CARTESIAN_POINT('',(52.,18.6896933872332,29.9768542348512)) ;
#13679=CARTESIAN_POINT('',(33.9,18.4371946053327,30.2293530167517)) ;
#13680=CARTESIAN_POINT('',(33.9,18.9592622740244,29.70728534806)) ;
#13681=CARTESIAN_POINT('',(70.1,18.4371946053327,30.2293530167517)) ;
#13682=CARTESIAN_POINT('',(52.,18.4371946053327,30.2293530167517)) ;
#13683=CARTESIAN_POINT('',(70.1,18.9592622740244,29.70728534806)) ;
#13684=CARTESIAN_POINT('Origin',(70.1,19.6310137161517,31.3689862838483)) ;
#13685=CARTESIAN_POINT('',(70.1,21.0231457651488,32.3103066127668)) ;
#13686=CARTESIAN_POINT('Origin',(70.1,25.5,25.5)) ;
#13687=CARTESIAN_POINT('',(70.1,20.7706469832483,32.5628053946673)) ;
#13688=CARTESIAN_POINT('Origin',(70.1,25.5,25.5)) ;
#13689=CARTESIAN_POINT('',(70.1,20.3027651582789,33.0306872196367)) ;
#13690=CARTESIAN_POINT('Origin',(33.9,21.29271465194,32.0407377259756)) ;
#13691=CARTESIAN_POINT('',(33.9,21.0231457651488,32.3103066127668)) ;
#13692=CARTESIAN_POINT('',(52.,21.0231457651488,32.3103066127668)) ;
#13693=CARTESIAN_POINT('',(33.9,20.7706469832483,32.5628053946673)) ;
#13694=CARTESIAN_POINT('',(52.,20.7706469832483,32.5628053946673)) ;
#13695=CARTESIAN_POINT('',(33.9,20.3027651582789,33.0306872196367)) ;
#13696=CARTESIAN_POINT('Origin',(33.9,19.6310137161517,31.3689862838483)) ;
#13697=CARTESIAN_POINT('Origin',(33.9,25.5,25.5)) ;
#13698=CARTESIAN_POINT('Origin',(33.9,25.5,25.5)) ;
#13699=CARTESIAN_POINT('Origin',(52.,25.5,25.5)) ;
#13700=CARTESIAN_POINT('',(71.,17.35,25.5)) ;
#13701=CARTESIAN_POINT('Origin',(71.,25.5,25.5)) ;
#13702=CARTESIAN_POINT('',(33.,17.35,25.5)) ;
#13703=CARTESIAN_POINT('',(52.,17.35,25.5)) ;
#13704=CARTESIAN_POINT('Origin',(33.,25.5,25.5)) ;
#13705=CARTESIAN_POINT('Origin',(33.,34.,25.5)) ;
#13706=CARTESIAN_POINT('',(33.,17.,25.5)) ;
#13707=CARTESIAN_POINT('Origin',(33.,25.5,25.5)) ;
#13708=CARTESIAN_POINT('Origin',(52.,25.5,25.5)) ;
#13709=CARTESIAN_POINT('',(71.,17.,25.5)) ;
#13710=CARTESIAN_POINT('Origin',(71.,25.5,25.5)) ;
#13711=CARTESIAN_POINT('',(52.,17.,25.5)) ;
#13712=CARTESIAN_POINT('Origin',(71.,33.65,25.5)) ;
#16928=UNCERTAINTY_MEASURE_WITH_UNIT(LENGTH_MEASURE(0.01),#16943,
'DISTANCE_ACCURACY_VALUE',
'Maximum model space distance between geometric entities at asserted c
onnectivities') ;
#16933=UNCERTAINTY_MEASURE_WITH_UNIT(LENGTH_MEASURE(0.01),#16943,
'DISTANCE_ACCURACY_VALUE',
'Maximum model space distance between geometric entities at asserted c
onnectivities') ;
#16937=(
GEOMETRIC_REPRESENTATION_CONTEXT(3)
GLOBAL_UNCERTAINTY_ASSIGNED_CONTEXT((#16928))
GLOBAL_UNIT_ASSIGNED_CONTEXT((#16943,#16945,#16946))
REPRESENTATION_CONTEXT('','3D')
) ;
#16942=(
GEOMETRIC_REPRESENTATION_CONTEXT(3)
GLOBAL_UNCERTAINTY_ASSIGNED_CONTEXT((#16933))
GLOBAL_UNIT_ASSIGNED_CONTEXT((#16943,#16945,#16946))
REPRESENTATION_CONTEXT('','3D')
) ;
#16943=(
LENGTH_UNIT()
NAMED_UNIT(*)
SI_UNIT(.MILLI.,.METRE.)
) ;
#16945=(
NAMED_UNIT(*)
PLANE_ANGLE_UNIT()
SI_UNIT($,.RADIAN.)
) ;
#16946=(
NAMED_UNIT(*)
SI_UNIT($,.STERADIAN.)
SOLID_ANGLE_UNIT()
) ;
#16950=SHAPE_DEFINITION_REPRESENTATION(#16958,#17021) ;
#16958=PRODUCT_DEFINITION_SHAPE('',$,#17030) ;
#17021=SHAPE_REPRESENTATION('',(#8552),#16937) ;
#17026=PRODUCT_DEFINITION_CONTEXT('part definition',#17052,'design') ;
#17030=PRODUCT_DEFINITION('Internal Ball Retainer Cage BSLM16',
'Internal Ball Retainer Cage BSLM16',#17038,#17026) ;
#17038=PRODUCT_DEFINITION_FORMATION('',$,#17057) ;
#17052=APPLICATION_CONTEXT(
'Core Data for Automotive Mechanical Design Process') ;
#17053=PRODUCT_CONTEXT('part definition',#17052,'mechanical') ;
#17057=PRODUCT('Internal Ball Retainer Cage BSLM16',
'Internal Ball Retainer Cage BSLM16',$,(#17053)) ;
#17065=PRESENTATION_STYLE_ASSIGNMENT((#17073)) ;
#17073=SURFACE_STYLE_USAGE(.BOTH.,#17081) ;
#17081=SURFACE_SIDE_STYLE('',(#17089)) ;
#17089=SURFACE_STYLE_FILL_AREA(#17097) ;
#17097=FILL_AREA_STYLE(
'MAS-257 Plastic - Internal Ball Retainer Cage BSLM16',(#17105)) ;
#17105=FILL_AREA_STYLE_COLOUR(
'MAS-257 Plastic - Internal Ball Retainer Cage BSLM16',#17113) ;
#17113=COLOUR_RGB(
'MAS-257 Plastic - Internal Ball Retainer Cage BSLM16', 0.40784314, 0.44705882, 0.49803922) ;
ENDSEC;
END-ISO-10303-21;
